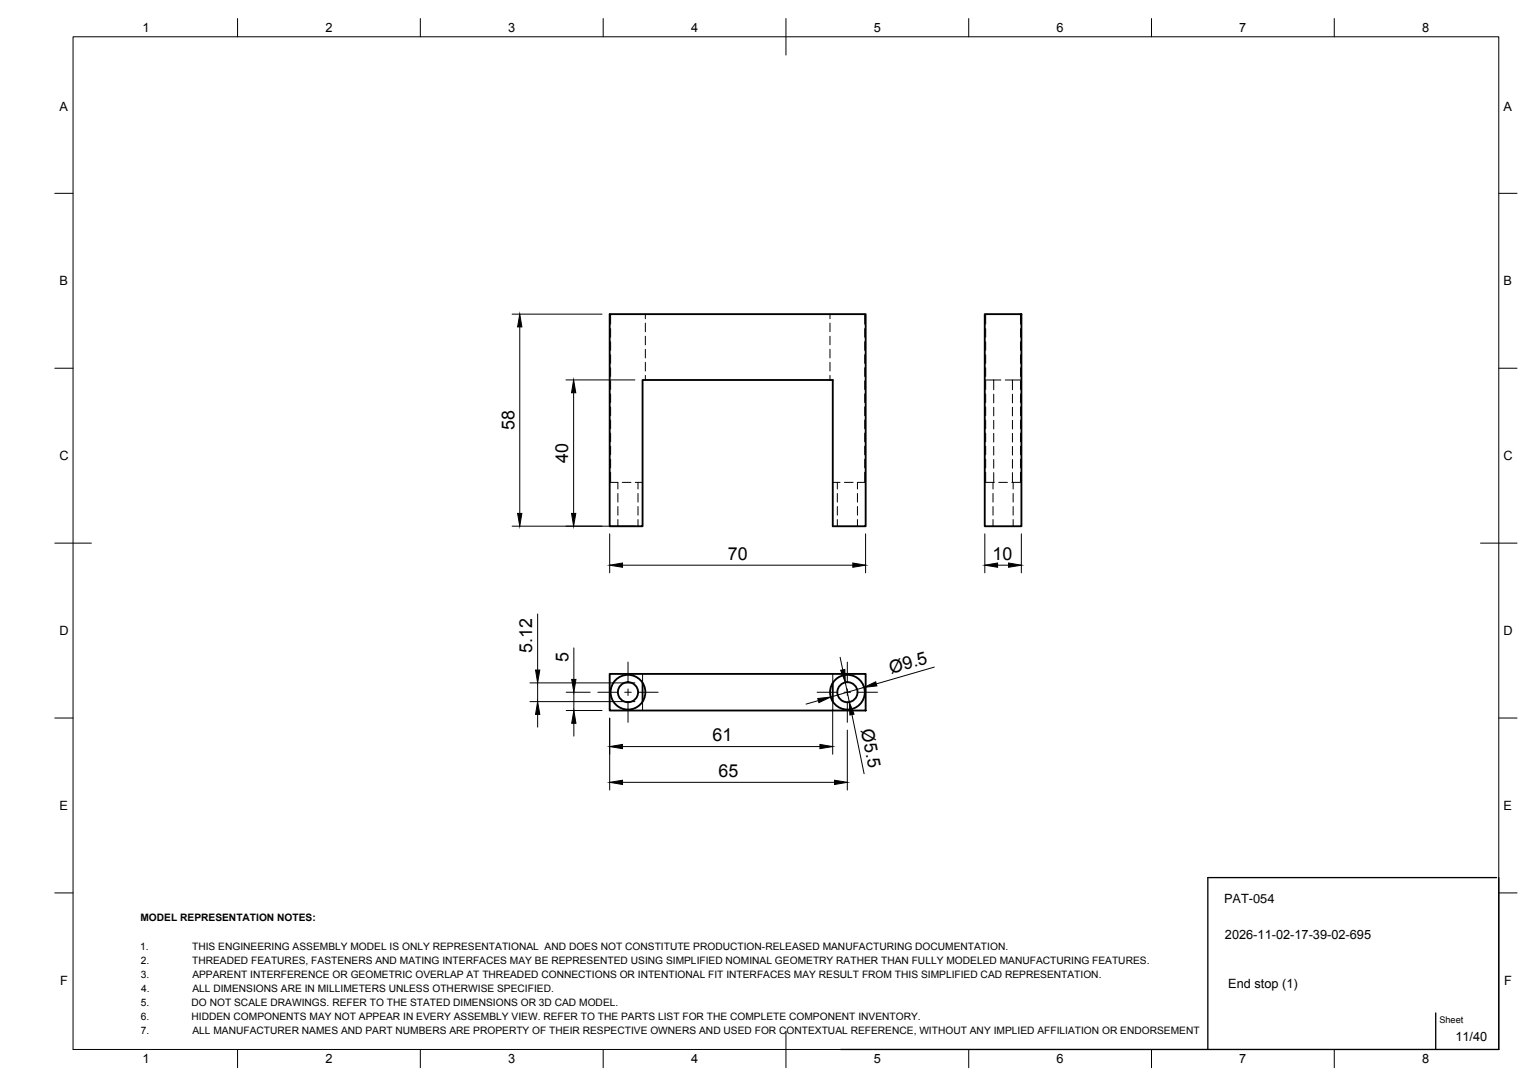
ISO-10303-21;
HEADER;
/* Generated by software containing ST-Developer
 * from STEP Tools, Inc. (www.steptools.com) 
 */

FILE_DESCRIPTION(
/* description */ ('PAT-054'),
/* implementation_level */ '2;1');

FILE_NAME(
/* name */ 'End stop (1).step',
/* time_stamp */ '2026-10-29T16:38:13-07:00',
/* author */ (''),
/* organization */ (''),
/* preprocessor_version */ 'ST-DEVELOPER v20.2',
/* originating_system */ 'Autodesk Translation Framework v15.17.0.0',
/* authorisation */ '');

FILE_SCHEMA (('AUTOMOTIVE_DESIGN { 1 0 10303 214 3 1 1 }'));
ENDSEC;

DATA;
#10=MECHANICAL_DESIGN_GEOMETRIC_PRESENTATION_REPRESENTATION('',(#906),#33981);
#818=SHAPE_REPRESENTATION_RELATIONSHIP('SRR','None',#34191,#862);
#862=ADVANCED_BREP_SHAPE_REPRESENTATION('',(#965),#33939);
#906=STYLED_ITEM('',(#34510),#965);
#965=MANIFOLD_SOLID_BREP('Body1',#13017);
#1110=FACE_BOUND('',#2508,.T.);
#1111=FACE_BOUND('',#2511,.T.);
#1112=FACE_BOUND('',#2520,.T.);
#1113=FACE_BOUND('',#2525,.T.);
#1114=FACE_BOUND('',#2526,.T.);
#1115=FACE_BOUND('',#2528,.T.);
#1281=PLANE('',#13800);
#1282=PLANE('',#13807);
#1283=PLANE('',#13814);
#1284=PLANE('',#13815);
#1285=PLANE('',#13820);
#1286=PLANE('',#13821);
#1287=PLANE('',#13822);
#1288=PLANE('',#13823);
#1289=PLANE('',#13824);
#1290=PLANE('',#13825);
#1291=PLANE('',#13826);
#1292=PLANE('',#13827);
#1686=FACE_OUTER_BOUND('',#2507,.T.);
#1687=FACE_OUTER_BOUND('',#2509,.T.);
#1688=FACE_OUTER_BOUND('',#2510,.T.);
#1689=FACE_OUTER_BOUND('',#2512,.T.);
#1690=FACE_OUTER_BOUND('',#2513,.T.);
#1691=FACE_OUTER_BOUND('',#2514,.T.);
#1692=FACE_OUTER_BOUND('',#2515,.T.);
#1693=FACE_OUTER_BOUND('',#2516,.T.);
#1694=FACE_OUTER_BOUND('',#2517,.T.);
#1695=FACE_OUTER_BOUND('',#2518,.T.);
#1696=FACE_OUTER_BOUND('',#2519,.T.);
#1697=FACE_OUTER_BOUND('',#2521,.T.);
#1698=FACE_OUTER_BOUND('',#2522,.T.);
#1699=FACE_OUTER_BOUND('',#2523,.T.);
#1700=FACE_OUTER_BOUND('',#2524,.T.);
#1701=FACE_OUTER_BOUND('',#2527,.T.);
#2507=EDGE_LOOP('',(#9011,#9012,#9013));
#2508=EDGE_LOOP('',(#9014));
#2509=EDGE_LOOP('',(#9015,#9016,#9017,#9018,#9019,#9020,#9021,#9022));
#2510=EDGE_LOOP('',(#9023,#9024,#9025));
#2511=EDGE_LOOP('',(#9026));
#2512=EDGE_LOOP('',(#9027,#9028,#9029,#9030,#9031,#9032,#9033,#9034));
#2513=EDGE_LOOP('',(#9035,#9036,#9037,#9038,#9039,#9040,#9041,#9042));
#2514=EDGE_LOOP('',(#9043,#9044,#9045,#9046,#9047,#9048,#9049,#9050));
#2515=EDGE_LOOP('',(#9051,#9052,#9053,#9054));
#2516=EDGE_LOOP('',(#9055,#9056,#9057,#9058));
#2517=EDGE_LOOP('',(#9059,#9060,#9061,#9062,#9063,#9064,#9065,#9066));
#2518=EDGE_LOOP('',(#9067,#9068,#9069,#9070,#9071,#9072,#9073,#9074));
#2519=EDGE_LOOP('',(#9075,#9076,#9077,#9078));
#2520=EDGE_LOOP('',(#9079));
#2521=EDGE_LOOP('',(#9080,#9081,#9082,#9083));
#2522=EDGE_LOOP('',(#9084,#9085,#9086,#9087));
#2523=EDGE_LOOP('',(#9088,#9089,#9090,#9091,#9092,#9093,#9094,#9095));
#2524=EDGE_LOOP('',(#9096,#9097,#9098,#9099));
#2525=EDGE_LOOP('',(#9100));
#2526=EDGE_LOOP('',(#9101));
#2527=EDGE_LOOP('',(#9102,#9103,#9104,#9105));
#2528=EDGE_LOOP('',(#9106));
#3378=LINE('',#19045,#4312);
#3379=LINE('',#19053,#4313);
#3380=LINE('',#19056,#4314);
#3381=LINE('',#19058,#4315);
#3382=LINE('',#19063,#4316);
#3383=LINE('',#19071,#4317);
#3384=LINE('',#19074,#4318);
#3385=LINE('',#19076,#4319);
#3386=LINE('',#19080,#4320);
#3387=LINE('',#19082,#4321);
#3388=LINE('',#19084,#4322);
#3389=LINE('',#19086,#4323);
#3390=LINE('',#19087,#4324);
#3391=LINE('',#19090,#4325);
#3392=LINE('',#19092,#4326);
#3393=LINE('',#19094,#4327);
#3394=LINE('',#19096,#4328);
#3395=LINE('',#19097,#4329);
#3396=LINE('',#19101,#4330);
#3397=LINE('',#19105,#4331);
#3398=LINE('',#19107,#4332);
#3399=LINE('',#19108,#4333);
#3400=LINE('',#19111,#4334);
#3401=LINE('',#19113,#4335);
#3402=LINE('',#19115,#4336);
#3403=LINE('',#19117,#4337);
#3404=LINE('',#19118,#4338);
#3405=LINE('',#19121,#4339);
#3406=LINE('',#19122,#4340);
#3407=LINE('',#19125,#4341);
#3408=LINE('',#19126,#4342);
#3409=LINE('',#19129,#4343);
#3410=LINE('',#19131,#4344);
#3411=LINE('',#19132,#4345);
#3412=LINE('',#19134,#4346);
#3413=LINE('',#19135,#4347);
#4312=VECTOR('',#15515,1.);
#4313=VECTOR('',#15524,1.);
#4314=VECTOR('',#15527,1.);
#4315=VECTOR('',#15528,0.475000000000001);
#4316=VECTOR('',#15533,1.);
#4317=VECTOR('',#15542,1.);
#4318=VECTOR('',#15545,1.);
#4319=VECTOR('',#15546,0.475000000000001);
#4320=VECTOR('',#15551,1.);
#4321=VECTOR('',#15552,1.);
#4322=VECTOR('',#15553,1.);
#4323=VECTOR('',#15554,1.);
#4324=VECTOR('',#15555,1.);
#4325=VECTOR('',#15558,1.);
#4326=VECTOR('',#15559,1.);
#4327=VECTOR('',#15560,1.);
#4328=VECTOR('',#15561,1.);
#4329=VECTOR('',#15562,1.);
#4330=VECTOR('',#15567,0.274999999999999);
#4331=VECTOR('',#15572,0.274999999999999);
#4332=VECTOR('',#15575,1.);
#4333=VECTOR('',#15576,1.);
#4334=VECTOR('',#15579,1.);
#4335=VECTOR('',#15580,1.);
#4336=VECTOR('',#15581,1.);
#4337=VECTOR('',#15582,1.);
#4338=VECTOR('',#15583,1.);
#4339=VECTOR('',#15586,1.);
#4340=VECTOR('',#15587,1.);
#4341=VECTOR('',#15590,1.);
#4342=VECTOR('',#15591,1.);
#4343=VECTOR('',#15594,1.);
#4344=VECTOR('',#15595,1.);
#4345=VECTOR('',#15596,1.);
#4346=VECTOR('',#15599,1.);
#4347=VECTOR('',#15600,1.);
#5225=CIRCLE('',#13801,0.475000000000001);
#5226=CIRCLE('',#13802,0.475000000000001);
#5227=CIRCLE('',#13803,0.274999999999999);
#5228=CIRCLE('',#13805,0.475000000000001);
#5229=CIRCLE('',#13806,0.475000000000001);
#5230=CIRCLE('',#13808,0.475000000000001);
#5231=CIRCLE('',#13809,0.475000000000001);
#5232=CIRCLE('',#13810,0.274999999999999);
#5233=CIRCLE('',#13812,0.475000000000001);
#5234=CIRCLE('',#13813,0.475000000000001);
#5235=CIRCLE('',#13817,0.274999999999999);
#5236=CIRCLE('',#13819,0.274999999999999);
#5744=VERTEX_POINT('',#19043);
#5745=VERTEX_POINT('',#19044);
#5746=VERTEX_POINT('',#19046);
#5747=VERTEX_POINT('',#19049);
#5748=VERTEX_POINT('',#19052);
#5749=VERTEX_POINT('',#19054);
#5750=VERTEX_POINT('',#19057);
#5751=VERTEX_POINT('',#19061);
#5752=VERTEX_POINT('',#19062);
#5753=VERTEX_POINT('',#19064);
#5754=VERTEX_POINT('',#19067);
#5755=VERTEX_POINT('',#19070);
#5756=VERTEX_POINT('',#19072);
#5757=VERTEX_POINT('',#19075);
#5758=VERTEX_POINT('',#19079);
#5759=VERTEX_POINT('',#19081);
#5760=VERTEX_POINT('',#19083);
#5761=VERTEX_POINT('',#19085);
#5762=VERTEX_POINT('',#19089);
#5763=VERTEX_POINT('',#19091);
#5764=VERTEX_POINT('',#19093);
#5765=VERTEX_POINT('',#19095);
#5766=VERTEX_POINT('',#19099);
#5767=VERTEX_POINT('',#19103);
#5768=VERTEX_POINT('',#19110);
#5769=VERTEX_POINT('',#19112);
#5770=VERTEX_POINT('',#19114);
#5771=VERTEX_POINT('',#19116);
#5772=VERTEX_POINT('',#19120);
#5773=VERTEX_POINT('',#19124);
#5774=VERTEX_POINT('',#19128);
#5775=VERTEX_POINT('',#19130);
#7005=EDGE_CURVE('',#5744,#5745,#3378,.T.);
#7006=EDGE_CURVE('',#5744,#5746,#5225,.T.);
#7007=EDGE_CURVE('',#5746,#5745,#5226,.T.);
#7008=EDGE_CURVE('',#5747,#5747,#5227,.T.);
#7009=EDGE_CURVE('',#5748,#5744,#3379,.T.);
#7010=EDGE_CURVE('',#5749,#5748,#5228,.T.);
#7011=EDGE_CURVE('',#5745,#5749,#3380,.T.);
#7012=EDGE_CURVE('',#5746,#5750,#3381,.T.);
#7013=EDGE_CURVE('',#5750,#5750,#5229,.T.);
#7014=EDGE_CURVE('',#5751,#5752,#3382,.T.);
#7015=EDGE_CURVE('',#5751,#5753,#5230,.T.);
#7016=EDGE_CURVE('',#5753,#5752,#5231,.T.);
#7017=EDGE_CURVE('',#5754,#5754,#5232,.T.);
#7018=EDGE_CURVE('',#5755,#5751,#3383,.T.);
#7019=EDGE_CURVE('',#5756,#5755,#5233,.T.);
#7020=EDGE_CURVE('',#5752,#5756,#3384,.T.);
#7021=EDGE_CURVE('',#5753,#5757,#3385,.T.);
#7022=EDGE_CURVE('',#5757,#5757,#5234,.T.);
#7023=EDGE_CURVE('',#5749,#5758,#3386,.T.);
#7024=EDGE_CURVE('',#5759,#5758,#3387,.T.);
#7025=EDGE_CURVE('',#5760,#5759,#3388,.T.);
#7026=EDGE_CURVE('',#5761,#5760,#3389,.T.);
#7027=EDGE_CURVE('',#5761,#5748,#3390,.T.);
#7028=EDGE_CURVE('',#5762,#5756,#3391,.T.);
#7029=EDGE_CURVE('',#5763,#5762,#3392,.T.);
#7030=EDGE_CURVE('',#5764,#5763,#3393,.T.);
#7031=EDGE_CURVE('',#5765,#5764,#3394,.T.);
#7032=EDGE_CURVE('',#5755,#5765,#3395,.T.);
#7033=EDGE_CURVE('',#5766,#5766,#5235,.T.);
#7034=EDGE_CURVE('',#5766,#5747,#3396,.T.);
#7035=EDGE_CURVE('',#5767,#5767,#5236,.T.);
#7036=EDGE_CURVE('',#5767,#5754,#3397,.T.);
#7037=EDGE_CURVE('',#5762,#5761,#3398,.T.);
#7038=EDGE_CURVE('',#5758,#5765,#3399,.T.);
#7039=EDGE_CURVE('',#5764,#5768,#3400,.T.);
#7040=EDGE_CURVE('',#5768,#5769,#3401,.T.);
#7041=EDGE_CURVE('',#5770,#5769,#3402,.T.);
#7042=EDGE_CURVE('',#5771,#5770,#3403,.T.);
#7043=EDGE_CURVE('',#5771,#5759,#3404,.T.);
#7044=EDGE_CURVE('',#5772,#5763,#3405,.T.);
#7045=EDGE_CURVE('',#5768,#5772,#3406,.T.);
#7046=EDGE_CURVE('',#5772,#5773,#3407,.T.);
#7047=EDGE_CURVE('',#5769,#5773,#3408,.T.);
#7048=EDGE_CURVE('',#5774,#5771,#3409,.T.);
#7049=EDGE_CURVE('',#5775,#5770,#3410,.T.);
#7050=EDGE_CURVE('',#5774,#5775,#3411,.T.);
#7051=EDGE_CURVE('',#5760,#5774,#3412,.T.);
#7052=EDGE_CURVE('',#5773,#5775,#3413,.T.);
#9011=ORIENTED_EDGE('',*,*,#7005,.F.);
#9012=ORIENTED_EDGE('',*,*,#7006,.T.);
#9013=ORIENTED_EDGE('',*,*,#7007,.T.);
#9014=ORIENTED_EDGE('',*,*,#7008,.F.);
#9015=ORIENTED_EDGE('',*,*,#7009,.F.);
#9016=ORIENTED_EDGE('',*,*,#7010,.F.);
#9017=ORIENTED_EDGE('',*,*,#7011,.F.);
#9018=ORIENTED_EDGE('',*,*,#7007,.F.);
#9019=ORIENTED_EDGE('',*,*,#7012,.T.);
#9020=ORIENTED_EDGE('',*,*,#7013,.F.);
#9021=ORIENTED_EDGE('',*,*,#7012,.F.);
#9022=ORIENTED_EDGE('',*,*,#7006,.F.);
#9023=ORIENTED_EDGE('',*,*,#7014,.F.);
#9024=ORIENTED_EDGE('',*,*,#7015,.T.);
#9025=ORIENTED_EDGE('',*,*,#7016,.T.);
#9026=ORIENTED_EDGE('',*,*,#7017,.F.);
#9027=ORIENTED_EDGE('',*,*,#7018,.F.);
#9028=ORIENTED_EDGE('',*,*,#7019,.F.);
#9029=ORIENTED_EDGE('',*,*,#7020,.F.);
#9030=ORIENTED_EDGE('',*,*,#7016,.F.);
#9031=ORIENTED_EDGE('',*,*,#7021,.T.);
#9032=ORIENTED_EDGE('',*,*,#7022,.F.);
#9033=ORIENTED_EDGE('',*,*,#7021,.F.);
#9034=ORIENTED_EDGE('',*,*,#7015,.F.);
#9035=ORIENTED_EDGE('',*,*,#7009,.T.);
#9036=ORIENTED_EDGE('',*,*,#7005,.T.);
#9037=ORIENTED_EDGE('',*,*,#7011,.T.);
#9038=ORIENTED_EDGE('',*,*,#7023,.T.);
#9039=ORIENTED_EDGE('',*,*,#7024,.F.);
#9040=ORIENTED_EDGE('',*,*,#7025,.F.);
#9041=ORIENTED_EDGE('',*,*,#7026,.F.);
#9042=ORIENTED_EDGE('',*,*,#7027,.T.);
#9043=ORIENTED_EDGE('',*,*,#7018,.T.);
#9044=ORIENTED_EDGE('',*,*,#7014,.T.);
#9045=ORIENTED_EDGE('',*,*,#7020,.T.);
#9046=ORIENTED_EDGE('',*,*,#7028,.F.);
#9047=ORIENTED_EDGE('',*,*,#7029,.F.);
#9048=ORIENTED_EDGE('',*,*,#7030,.F.);
#9049=ORIENTED_EDGE('',*,*,#7031,.F.);
#9050=ORIENTED_EDGE('',*,*,#7032,.F.);
#9051=ORIENTED_EDGE('',*,*,#7033,.F.);
#9052=ORIENTED_EDGE('',*,*,#7034,.T.);
#9053=ORIENTED_EDGE('',*,*,#7008,.T.);
#9054=ORIENTED_EDGE('',*,*,#7034,.F.);
#9055=ORIENTED_EDGE('',*,*,#7035,.F.);
#9056=ORIENTED_EDGE('',*,*,#7036,.T.);
#9057=ORIENTED_EDGE('',*,*,#7017,.T.);
#9058=ORIENTED_EDGE('',*,*,#7036,.F.);
#9059=ORIENTED_EDGE('',*,*,#7010,.T.);
#9060=ORIENTED_EDGE('',*,*,#7027,.F.);
#9061=ORIENTED_EDGE('',*,*,#7037,.F.);
#9062=ORIENTED_EDGE('',*,*,#7028,.T.);
#9063=ORIENTED_EDGE('',*,*,#7019,.T.);
#9064=ORIENTED_EDGE('',*,*,#7032,.T.);
#9065=ORIENTED_EDGE('',*,*,#7038,.F.);
#9066=ORIENTED_EDGE('',*,*,#7023,.F.);
#9067=ORIENTED_EDGE('',*,*,#7024,.T.);
#9068=ORIENTED_EDGE('',*,*,#7038,.T.);
#9069=ORIENTED_EDGE('',*,*,#7031,.T.);
#9070=ORIENTED_EDGE('',*,*,#7039,.T.);
#9071=ORIENTED_EDGE('',*,*,#7040,.T.);
#9072=ORIENTED_EDGE('',*,*,#7041,.F.);
#9073=ORIENTED_EDGE('',*,*,#7042,.F.);
#9074=ORIENTED_EDGE('',*,*,#7043,.T.);
#9075=ORIENTED_EDGE('',*,*,#7030,.T.);
#9076=ORIENTED_EDGE('',*,*,#7044,.F.);
#9077=ORIENTED_EDGE('',*,*,#7045,.F.);
#9078=ORIENTED_EDGE('',*,*,#7039,.F.);
#9079=ORIENTED_EDGE('',*,*,#7035,.T.);
#9080=ORIENTED_EDGE('',*,*,#7045,.T.);
#9081=ORIENTED_EDGE('',*,*,#7046,.T.);
#9082=ORIENTED_EDGE('',*,*,#7047,.F.);
#9083=ORIENTED_EDGE('',*,*,#7040,.F.);
#9084=ORIENTED_EDGE('',*,*,#7048,.T.);
#9085=ORIENTED_EDGE('',*,*,#7042,.T.);
#9086=ORIENTED_EDGE('',*,*,#7049,.F.);
#9087=ORIENTED_EDGE('',*,*,#7050,.F.);
#9088=ORIENTED_EDGE('',*,*,#7026,.T.);
#9089=ORIENTED_EDGE('',*,*,#7051,.T.);
#9090=ORIENTED_EDGE('',*,*,#7050,.T.);
#9091=ORIENTED_EDGE('',*,*,#7052,.F.);
#9092=ORIENTED_EDGE('',*,*,#7046,.F.);
#9093=ORIENTED_EDGE('',*,*,#7044,.T.);
#9094=ORIENTED_EDGE('',*,*,#7029,.T.);
#9095=ORIENTED_EDGE('',*,*,#7037,.T.);
#9096=ORIENTED_EDGE('',*,*,#7052,.T.);
#9097=ORIENTED_EDGE('',*,*,#7049,.T.);
#9098=ORIENTED_EDGE('',*,*,#7041,.T.);
#9099=ORIENTED_EDGE('',*,*,#7047,.T.);
#9100=ORIENTED_EDGE('',*,*,#7013,.T.);
#9101=ORIENTED_EDGE('',*,*,#7022,.T.);
#9102=ORIENTED_EDGE('',*,*,#7025,.T.);
#9103=ORIENTED_EDGE('',*,*,#7043,.F.);
#9104=ORIENTED_EDGE('',*,*,#7048,.F.);
#9105=ORIENTED_EDGE('',*,*,#7051,.F.);
#9106=ORIENTED_EDGE('',*,*,#7033,.T.);
#12037=CYLINDRICAL_SURFACE('',#13804,0.475000000000001);
#12038=CYLINDRICAL_SURFACE('',#13811,0.475000000000001);
#12039=CYLINDRICAL_SURFACE('',#13816,0.274999999999999);
#12040=CYLINDRICAL_SURFACE('',#13818,0.274999999999999);
#12398=ADVANCED_FACE('',(#1686,#1110),#1281,.T.);
#12399=ADVANCED_FACE('',(#1687),#12037,.F.);
#12400=ADVANCED_FACE('',(#1688,#1111),#1282,.T.);
#12401=ADVANCED_FACE('',(#1689),#12038,.F.);
#12402=ADVANCED_FACE('',(#1690),#1283,.F.);
#12403=ADVANCED_FACE('',(#1691),#1284,.F.);
#12404=ADVANCED_FACE('',(#1692),#12039,.F.);
#12405=ADVANCED_FACE('',(#1693),#12040,.F.);
#12406=ADVANCED_FACE('',(#1694),#1285,.F.);
#12407=ADVANCED_FACE('',(#1695),#1286,.T.);
#12408=ADVANCED_FACE('',(#1696,#1112),#1287,.F.);
#12409=ADVANCED_FACE('',(#1697),#1288,.T.);
#12410=ADVANCED_FACE('',(#1698),#1289,.T.);
#12411=ADVANCED_FACE('',(#1699),#1290,.T.);
#12412=ADVANCED_FACE('',(#1700,#1113,#1114),#1291,.T.);
#12413=ADVANCED_FACE('',(#1701,#1115),#1292,.F.);
#13017=CLOSED_SHELL('',(#12398,#12399,#12400,#12401,#12402,#12403,#12404,
#12405,#12406,#12407,#12408,#12409,#12410,#12411,#12412,#12413));
#13799=AXIS2_PLACEMENT_3D('',#19041,#15511,#15512);
#13800=AXIS2_PLACEMENT_3D('',#19042,#15513,#15514);
#13801=AXIS2_PLACEMENT_3D('',#19047,#15516,#15517);
#13802=AXIS2_PLACEMENT_3D('',#19048,#15518,#15519);
#13803=AXIS2_PLACEMENT_3D('',#19050,#15520,#15521);
#13804=AXIS2_PLACEMENT_3D('',#19051,#15522,#15523);
#13805=AXIS2_PLACEMENT_3D('',#19055,#15525,#15526);
#13806=AXIS2_PLACEMENT_3D('',#19059,#15529,#15530);
#13807=AXIS2_PLACEMENT_3D('',#19060,#15531,#15532);
#13808=AXIS2_PLACEMENT_3D('',#19065,#15534,#15535);
#13809=AXIS2_PLACEMENT_3D('',#19066,#15536,#15537);
#13810=AXIS2_PLACEMENT_3D('',#19068,#15538,#15539);
#13811=AXIS2_PLACEMENT_3D('',#19069,#15540,#15541);
#13812=AXIS2_PLACEMENT_3D('',#19073,#15543,#15544);
#13813=AXIS2_PLACEMENT_3D('',#19077,#15547,#15548);
#13814=AXIS2_PLACEMENT_3D('',#19078,#15549,#15550);
#13815=AXIS2_PLACEMENT_3D('',#19088,#15556,#15557);
#13816=AXIS2_PLACEMENT_3D('',#19098,#15563,#15564);
#13817=AXIS2_PLACEMENT_3D('',#19100,#15565,#15566);
#13818=AXIS2_PLACEMENT_3D('',#19102,#15568,#15569);
#13819=AXIS2_PLACEMENT_3D('',#19104,#15570,#15571);
#13820=AXIS2_PLACEMENT_3D('',#19106,#15573,#15574);
#13821=AXIS2_PLACEMENT_3D('',#19109,#15577,#15578);
#13822=AXIS2_PLACEMENT_3D('',#19119,#15584,#15585);
#13823=AXIS2_PLACEMENT_3D('',#19123,#15588,#15589);
#13824=AXIS2_PLACEMENT_3D('',#19127,#15592,#15593);
#13825=AXIS2_PLACEMENT_3D('',#19133,#15597,#15598);
#13826=AXIS2_PLACEMENT_3D('',#19136,#15601,#15602);
#13827=AXIS2_PLACEMENT_3D('',#19137,#15603,#15604);
#15511=DIRECTION('axis',(0.,0.,1.));
#15512=DIRECTION('refdir',(1.,0.,0.));
#15513=DIRECTION('center_axis',(0.,0.,1.));
#15514=DIRECTION('ref_axis',(1.,0.,0.));
#15515=DIRECTION('',(1.,0.,0.));
#15516=DIRECTION('center_axis',(0.,0.,1.));
#15517=DIRECTION('ref_axis',(1.,0.,0.));
#15518=DIRECTION('center_axis',(0.,0.,1.));
#15519=DIRECTION('ref_axis',(1.,0.,0.));
#15520=DIRECTION('center_axis',(0.,0.,1.));
#15521=DIRECTION('ref_axis',(1.,0.,0.));
#15522=DIRECTION('center_axis',(0.,0.,1.));
#15523=DIRECTION('ref_axis',(1.,0.,0.));
#15524=DIRECTION('',(0.,0.,-1.));
#15525=DIRECTION('center_axis',(0.,0.,1.));
#15526=DIRECTION('ref_axis',(1.,0.,0.));
#15527=DIRECTION('',(0.,0.,1.));
#15528=DIRECTION('',(0.,0.,1.));
#15529=DIRECTION('center_axis',(0.,0.,-1.));
#15530=DIRECTION('ref_axis',(1.,0.,0.));
#15531=DIRECTION('center_axis',(0.,0.,1.));
#15532=DIRECTION('ref_axis',(1.,0.,0.));
#15533=DIRECTION('',(-1.,0.,0.));
#15534=DIRECTION('center_axis',(0.,0.,1.));
#15535=DIRECTION('ref_axis',(1.,0.,0.));
#15536=DIRECTION('center_axis',(0.,0.,1.));
#15537=DIRECTION('ref_axis',(1.,0.,0.));
#15538=DIRECTION('center_axis',(0.,0.,1.));
#15539=DIRECTION('ref_axis',(1.,0.,0.));
#15540=DIRECTION('center_axis',(0.,0.,1.));
#15541=DIRECTION('ref_axis',(1.,0.,0.));
#15542=DIRECTION('',(0.,0.,-1.));
#15543=DIRECTION('center_axis',(0.,0.,1.));
#15544=DIRECTION('ref_axis',(1.,0.,0.));
#15545=DIRECTION('',(0.,0.,1.));
#15546=DIRECTION('',(0.,0.,1.));
#15547=DIRECTION('center_axis',(0.,0.,-1.));
#15548=DIRECTION('ref_axis',(1.,0.,0.));
#15549=DIRECTION('center_axis',(0.,-1.,0.));
#15550=DIRECTION('ref_axis',(0.,0.,-1.));
#15551=DIRECTION('',(1.,0.,0.));
#15552=DIRECTION('',(0.,0.,1.));
#15553=DIRECTION('',(1.,0.,0.));
#15554=DIRECTION('',(0.,0.,-1.));
#15555=DIRECTION('',(1.,0.,0.));
#15556=DIRECTION('center_axis',(0.,1.,0.));
#15557=DIRECTION('ref_axis',(0.,0.,1.));
#15558=DIRECTION('',(1.,0.,0.));
#15559=DIRECTION('',(0.,0.,1.));
#15560=DIRECTION('',(-1.,0.,0.));
#15561=DIRECTION('',(0.,0.,-1.));
#15562=DIRECTION('',(1.,0.,0.));
#15563=DIRECTION('center_axis',(0.,0.,1.));
#15564=DIRECTION('ref_axis',(1.,0.,0.));
#15565=DIRECTION('center_axis',(0.,0.,1.));
#15566=DIRECTION('ref_axis',(1.,0.,0.));
#15567=DIRECTION('',(0.,0.,1.));
#15568=DIRECTION('center_axis',(0.,0.,1.));
#15569=DIRECTION('ref_axis',(1.,0.,0.));
#15570=DIRECTION('center_axis',(0.,0.,1.));
#15571=DIRECTION('ref_axis',(1.,0.,0.));
#15572=DIRECTION('',(0.,0.,1.));
#15573=DIRECTION('center_axis',(0.,0.,1.));
#15574=DIRECTION('ref_axis',(0.,-1.,0.));
#15575=DIRECTION('',(0.,-1.,0.));
#15576=DIRECTION('',(0.,1.,0.));
#15577=DIRECTION('center_axis',(1.,0.,0.));
#15578=DIRECTION('ref_axis',(0.,1.,0.));
#15579=DIRECTION('',(0.,1.,0.));
#15580=DIRECTION('',(0.,0.,1.));
#15581=DIRECTION('',(0.,1.,0.));
#15582=DIRECTION('',(0.,0.,1.));
#15583=DIRECTION('',(0.,1.,0.));
#15584=DIRECTION('center_axis',(0.,0.,1.));
#15585=DIRECTION('ref_axis',(1.,0.,0.));
#15586=DIRECTION('',(0.,-1.,0.));
#15587=DIRECTION('',(-1.,0.,0.));
#15588=DIRECTION('center_axis',(0.,1.,0.));
#15589=DIRECTION('ref_axis',(-1.,0.,0.));
#15590=DIRECTION('',(0.,0.,1.));
#15591=DIRECTION('',(-1.,0.,0.));
#15592=DIRECTION('center_axis',(0.,-1.,0.));
#15593=DIRECTION('ref_axis',(1.,0.,0.));
#15594=DIRECTION('',(1.,0.,0.));
#15595=DIRECTION('',(1.,0.,0.));
#15596=DIRECTION('',(0.,0.,1.));
#15597=DIRECTION('center_axis',(-1.,0.,0.));
#15598=DIRECTION('ref_axis',(0.,-1.,0.));
#15599=DIRECTION('',(0.,-1.,0.));
#15600=DIRECTION('',(0.,-1.,0.));
#15601=DIRECTION('center_axis',(0.,0.,1.));
#15602=DIRECTION('ref_axis',(1.,0.,0.));
#15603=DIRECTION('center_axis',(0.,0.,1.));
#15604=DIRECTION('ref_axis',(1.,0.,0.));
#19041=CARTESIAN_POINT('',(0.,0.,0.));
#19042=CARTESIAN_POINT('Origin',(22.3,-9.,2.4));
#19043=CARTESIAN_POINT('',(22.043826230851,-8.6,2.4));
#19044=CARTESIAN_POINT('',(22.556173769149,-8.6,2.4));
#19045=CARTESIAN_POINT('',(22.,-8.6,2.4));
#19046=CARTESIAN_POINT('',(21.825,-9.,2.4));
#19047=CARTESIAN_POINT('Origin',(22.3,-9.,2.4));
#19048=CARTESIAN_POINT('Origin',(22.3,-9.,2.4));
#19049=CARTESIAN_POINT('',(22.025,-9.,2.4));
#19050=CARTESIAN_POINT('Origin',(22.3,-9.,2.4));
#19051=CARTESIAN_POINT('Origin',(22.3,-9.,2.4));
#19052=CARTESIAN_POINT('',(22.043826230851,-8.6,5.2));
#19053=CARTESIAN_POINT('',(22.043826230851,-8.6,2.4));
#19054=CARTESIAN_POINT('',(22.556173769149,-8.6,5.2));
#19055=CARTESIAN_POINT('Origin',(22.3,-9.,5.2));
#19056=CARTESIAN_POINT('',(22.556173769149,-8.6,2.4));
#19057=CARTESIAN_POINT('',(21.825,-9.,7.));
#19058=CARTESIAN_POINT('',(21.825,-9.,2.4));
#19059=CARTESIAN_POINT('Origin',(22.3,-9.,7.));
#19060=CARTESIAN_POINT('Origin',(22.3,-3.,2.4));
#19061=CARTESIAN_POINT('',(22.556173769149,-3.4,2.4));
#19062=CARTESIAN_POINT('',(22.043826230851,-3.4,2.4));
#19063=CARTESIAN_POINT('',(22.,-3.4,2.4));
#19064=CARTESIAN_POINT('',(21.825,-3.,2.4));
#19065=CARTESIAN_POINT('Origin',(22.3,-3.,2.4));
#19066=CARTESIAN_POINT('Origin',(22.3,-3.,2.4));
#19067=CARTESIAN_POINT('',(22.025,-3.,2.4));
#19068=CARTESIAN_POINT('Origin',(22.3,-3.,2.4));
#19069=CARTESIAN_POINT('Origin',(22.3,-3.,2.4));
#19070=CARTESIAN_POINT('',(22.556173769149,-3.4,5.2));
#19071=CARTESIAN_POINT('',(22.556173769149,-3.4,2.4));
#19072=CARTESIAN_POINT('',(22.043826230851,-3.4,5.2));
#19073=CARTESIAN_POINT('Origin',(22.3,-3.,5.2));
#19074=CARTESIAN_POINT('',(22.043826230851,-3.4,2.4));
#19075=CARTESIAN_POINT('',(21.825,-3.,7.));
#19076=CARTESIAN_POINT('',(21.825,-3.,2.4));
#19077=CARTESIAN_POINT('Origin',(22.3,-3.,7.));
#19078=CARTESIAN_POINT('Origin',(21.7,-8.6,5.2));
#19079=CARTESIAN_POINT('',(22.8,-8.6,5.2));
#19080=CARTESIAN_POINT('',(21.7,-8.6,5.2));
#19081=CARTESIAN_POINT('',(22.8,-8.6,1.2));
#19082=CARTESIAN_POINT('',(22.8,-8.6,3.2));
#19083=CARTESIAN_POINT('',(21.8,-8.6,1.2));
#19084=CARTESIAN_POINT('',(22.,-8.6,1.2));
#19085=CARTESIAN_POINT('',(21.8,-8.6,5.2));
#19086=CARTESIAN_POINT('',(21.8,-8.6,3.2));
#19087=CARTESIAN_POINT('',(21.7,-8.6,5.2));
#19088=CARTESIAN_POINT('Origin',(21.7,-3.4,1.2));
#19089=CARTESIAN_POINT('',(21.8,-3.4,5.2));
#19090=CARTESIAN_POINT('',(21.7,-3.4,5.2));
#19091=CARTESIAN_POINT('',(21.8,-3.4,1.2));
#19092=CARTESIAN_POINT('',(21.8,-3.4,1.2));
#19093=CARTESIAN_POINT('',(22.8,-3.4,1.2));
#19094=CARTESIAN_POINT('',(22.,-3.4,1.2));
#19095=CARTESIAN_POINT('',(22.8,-3.4,5.2));
#19096=CARTESIAN_POINT('',(22.8,-3.4,1.2));
#19097=CARTESIAN_POINT('',(21.7,-3.4,5.2));
#19098=CARTESIAN_POINT('Origin',(22.3,-9.,1.1));
#19099=CARTESIAN_POINT('',(22.025,-9.,1.2));
#19100=CARTESIAN_POINT('Origin',(22.3,-9.,1.2));
#19101=CARTESIAN_POINT('',(22.025,-9.,1.1));
#19102=CARTESIAN_POINT('Origin',(22.3,-3.,1.1));
#19103=CARTESIAN_POINT('',(22.025,-3.,1.2));
#19104=CARTESIAN_POINT('Origin',(22.3,-3.,1.2));
#19105=CARTESIAN_POINT('',(22.025,-3.,1.1));
#19106=CARTESIAN_POINT('Origin',(21.7,-3.4,5.2));
#19107=CARTESIAN_POINT('',(21.8,-2.95,5.2));
#19108=CARTESIAN_POINT('',(22.8,-6.45,5.2));
#19109=CARTESIAN_POINT('Origin',(22.8,-9.5,1.2));
#19110=CARTESIAN_POINT('',(22.8,-2.5,1.2));
#19111=CARTESIAN_POINT('',(22.8,-9.5,1.2));
#19112=CARTESIAN_POINT('',(22.8,-2.5,7.));
#19113=CARTESIAN_POINT('',(22.8,-2.5,1.2));
#19114=CARTESIAN_POINT('',(22.8,-9.5,7.));
#19115=CARTESIAN_POINT('',(22.8,-9.5,7.));
#19116=CARTESIAN_POINT('',(22.8,-9.5,1.2));
#19117=CARTESIAN_POINT('',(22.8,-9.5,1.2));
#19118=CARTESIAN_POINT('',(22.8,-9.5,1.2));
#19119=CARTESIAN_POINT('Origin',(22.3,-6.,1.2));
#19120=CARTESIAN_POINT('',(21.8,-2.5,1.2));
#19121=CARTESIAN_POINT('',(21.8,-2.5,1.2));
#19122=CARTESIAN_POINT('',(22.8,-2.5,1.2));
#19123=CARTESIAN_POINT('Origin',(22.8,-2.5,1.2));
#19124=CARTESIAN_POINT('',(21.8,-2.5,7.));
#19125=CARTESIAN_POINT('',(21.8,-2.5,1.2));
#19126=CARTESIAN_POINT('',(22.8,-2.5,7.));
#19127=CARTESIAN_POINT('Origin',(21.8,-9.5,1.2));
#19128=CARTESIAN_POINT('',(21.8,-9.5,1.2));
#19129=CARTESIAN_POINT('',(21.8,-9.5,1.2));
#19130=CARTESIAN_POINT('',(21.8,-9.5,7.));
#19131=CARTESIAN_POINT('',(21.8,-9.5,7.));
#19132=CARTESIAN_POINT('',(21.8,-9.5,1.2));
#19133=CARTESIAN_POINT('Origin',(21.8,-2.5,1.2));
#19134=CARTESIAN_POINT('',(21.8,-2.5,1.2));
#19135=CARTESIAN_POINT('',(21.8,-2.5,7.));
#19136=CARTESIAN_POINT('Origin',(22.3,-6.,7.));
#19137=CARTESIAN_POINT('Origin',(22.3,-6.,1.2));
#33887=UNCERTAINTY_MEASURE_WITH_UNIT(LENGTH_MEASURE(0.001),#33982,
'DISTANCE_ACCURACY_VALUE',
'Maximum model space distance between geometric entities at asserted c
onnectivities');
#33929=UNCERTAINTY_MEASURE_WITH_UNIT(LENGTH_MEASURE(0.001),#33982,
'DISTANCE_ACCURACY_VALUE',
'Maximum model space distance between geometric entities at asserted c
onnectivities');
#33939=(
GEOMETRIC_REPRESENTATION_CONTEXT(3)
GLOBAL_UNCERTAINTY_ASSIGNED_CONTEXT((#33887))
GLOBAL_UNIT_ASSIGNED_CONTEXT((#33982,#33984,#33985))
REPRESENTATION_CONTEXT('','3D')
);
#33981=(
GEOMETRIC_REPRESENTATION_CONTEXT(3)
GLOBAL_UNCERTAINTY_ASSIGNED_CONTEXT((#33929))
GLOBAL_UNIT_ASSIGNED_CONTEXT((#33982,#33984,#33985))
REPRESENTATION_CONTEXT('','3D')
);
#33982=(
LENGTH_UNIT()
NAMED_UNIT(*)
SI_UNIT(.CENTI.,.METRE.)
);
#33984=(
NAMED_UNIT(*)
PLANE_ANGLE_UNIT()
SI_UNIT($,.RADIAN.)
);
#33985=(
NAMED_UNIT(*)
SI_UNIT($,.STERADIAN.)
SOLID_ANGLE_UNIT()
);
#33995=SHAPE_DEFINITION_REPRESENTATION(#34046,#34191);
#34046=PRODUCT_DEFINITION_SHAPE('',$,#34243);
#34191=SHAPE_REPRESENTATION('',(#13799),#33939);
#34233=PRODUCT_DEFINITION_CONTEXT('part definition',#34388,'design');
#34243=PRODUCT_DEFINITION('End stop (1)','End stop (1)',#34294,#34233);
#34294=PRODUCT_DEFINITION_FORMATION('',$,#34399);
#34388=APPLICATION_CONTEXT(
'Core Data for Automotive Mechanical Design Process');
#34389=PRODUCT_CONTEXT('part definition',#34388,'mechanical');
#34399=PRODUCT('End stop (1)','End stop (1)','End stop (1)',(#34389));
#34504=COLOUR_RGB('Sky Blue',0.24,0.69,0.87);
#34505=FILL_AREA_STYLE_COLOUR('',#34504);
#34506=FILL_AREA_STYLE('',(#34505));
#34507=SURFACE_STYLE_FILL_AREA(#34506);
#34508=SURFACE_SIDE_STYLE('',(#34507));
#34509=SURFACE_STYLE_USAGE(.BOTH.,#34508);
#34510=PRESENTATION_STYLE_ASSIGNMENT((#34509));
ENDSEC;
END-ISO-10303-21;
